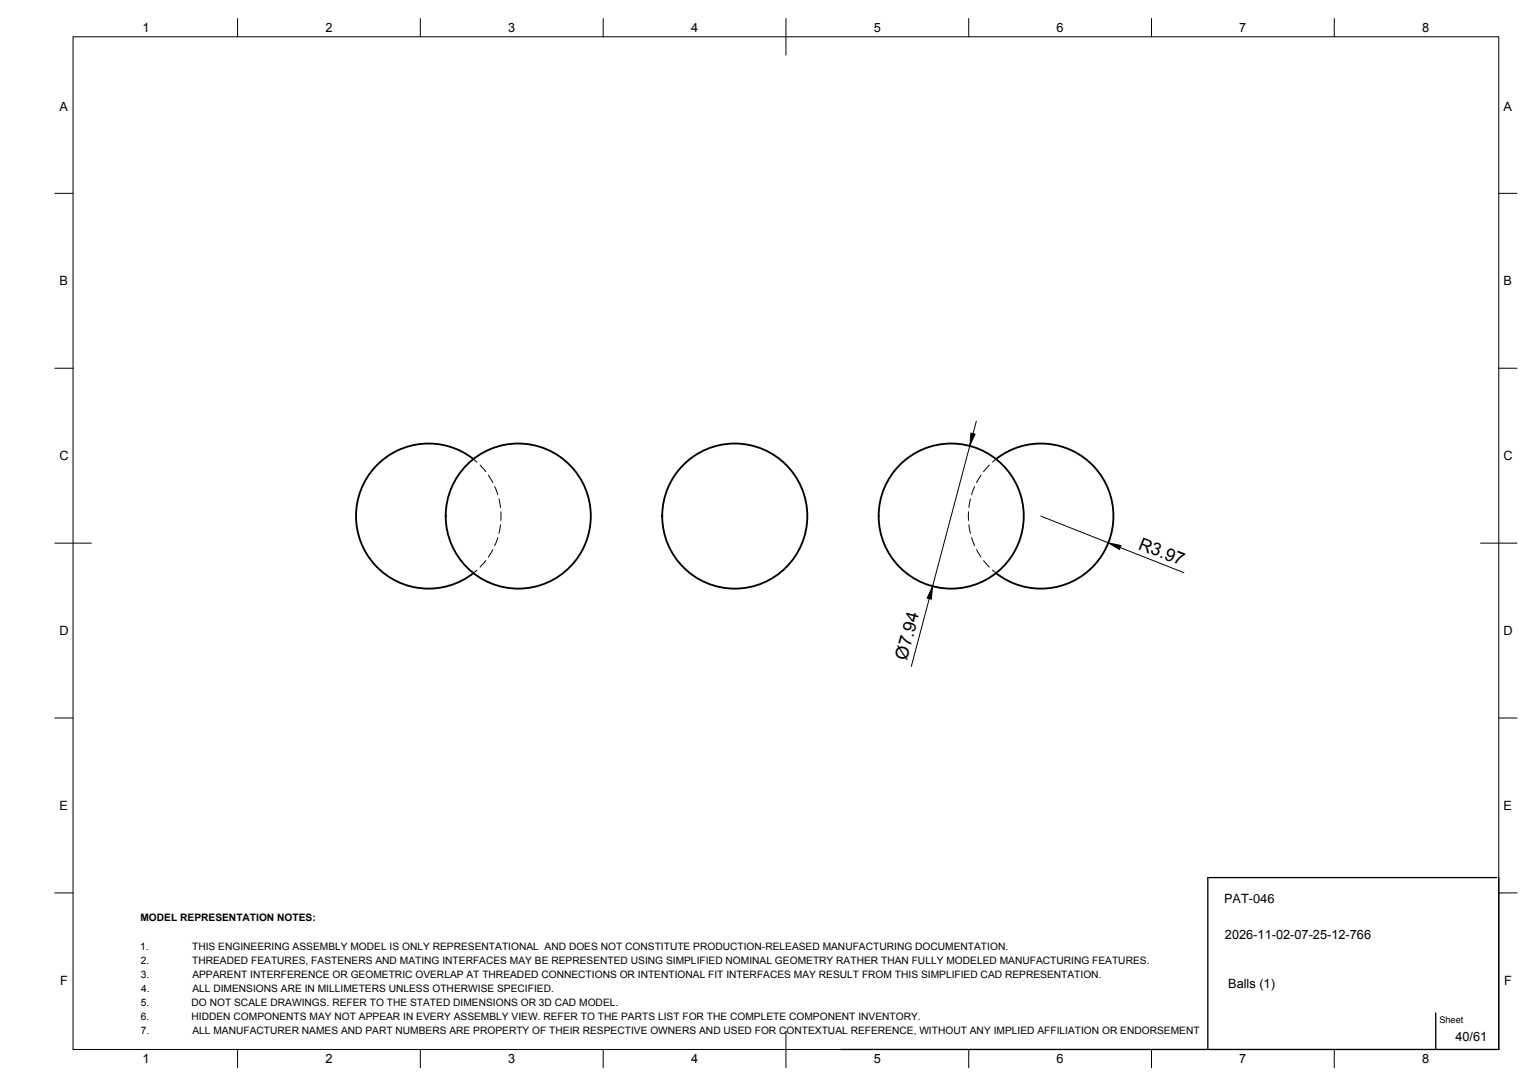
ISO-10303-21;
HEADER;
/* Generated by software containing ST-Developer
 * from STEP Tools, Inc. (www.steptools.com) 
 */

FILE_DESCRIPTION(
/* description */ ('Gear mesh backlash fixture'),
/* implementation_level */ '2;1');

FILE_NAME(
/* name */ 'Balls (1).step',
/* time_stamp */ '2026-10-28T03:26:00-07:00',
/* author */ (''),
/* organization */ (''),
/* preprocessor_version */ 'ST-DEVELOPER v20.2',
/* originating_system */ 'Autodesk Translation Framework v15.17.0.0',
/* authorisation */ '');

FILE_SCHEMA (('AUTOMOTIVE_DESIGN { 1 0 10303 214 3 1 1 }'));
ENDSEC;

DATA;
#10=MECHANICAL_DESIGN_GEOMETRIC_PRESENTATION_REPRESENTATION('',(#1053,#1054,#1055,#1056,#1057,#1058,#1059,#1060),#57900);
#743=SPHERICAL_SURFACE('',#14949,0.3969);
#744=SPHERICAL_SURFACE('',#14951,0.3969);
#745=SPHERICAL_SURFACE('',#14953,0.3969);
#746=SPHERICAL_SURFACE('',#14955,0.3969);
#747=SPHERICAL_SURFACE('',#14957,0.3969);
#748=SPHERICAL_SURFACE('',#14959,0.3969);
#749=SPHERICAL_SURFACE('',#14961,0.3969);
#750=SPHERICAL_SURFACE('',#14963,0.3969);
#946=SHAPE_REPRESENTATION_RELATIONSHIP('SRR','None',#58145,#996);
#996=ADVANCED_BREP_SHAPE_REPRESENTATION('',(#1116,#1117,#1118,#1119,#1120,
#1121,#1122,#1123),#57878);
#1053=STYLED_ITEM('',(#58465),#1116);
#1054=STYLED_ITEM('',(#58465),#1117);
#1055=STYLED_ITEM('',(#58465),#1118);
#1056=STYLED_ITEM('',(#58465),#1119);
#1057=STYLED_ITEM('',(#58465),#1120);
#1058=STYLED_ITEM('',(#58465),#1121);
#1059=STYLED_ITEM('',(#58465),#1122);
#1060=STYLED_ITEM('',(#58465),#1123);
#1116=MANIFOLD_SOLID_BREP('Body1',#13615);
#1117=MANIFOLD_SOLID_BREP('Body2',#13616);
#1118=MANIFOLD_SOLID_BREP('Body3',#13617);
#1119=MANIFOLD_SOLID_BREP('Body4',#13618);
#1120=MANIFOLD_SOLID_BREP('Body5',#13619);
#1121=MANIFOLD_SOLID_BREP('Body6',#13620);
#1122=MANIFOLD_SOLID_BREP('Body7',#13621);
#1123=MANIFOLD_SOLID_BREP('Body8',#13622);
#2060=FACE_OUTER_BOUND('',#2968,.T.);
#2061=FACE_OUTER_BOUND('',#2969,.T.);
#2062=FACE_OUTER_BOUND('',#2970,.T.);
#2063=FACE_OUTER_BOUND('',#2971,.T.);
#2064=FACE_OUTER_BOUND('',#2972,.T.);
#2065=FACE_OUTER_BOUND('',#2973,.T.);
#2066=FACE_OUTER_BOUND('',#2974,.T.);
#2067=FACE_OUTER_BOUND('',#2975,.T.);
#2968=EDGE_LOOP('',(#10539,#10540));
#2969=EDGE_LOOP('',(#10541,#10542));
#2970=EDGE_LOOP('',(#10543,#10544));
#2971=EDGE_LOOP('',(#10545,#10546));
#2972=EDGE_LOOP('',(#10547,#10548));
#2973=EDGE_LOOP('',(#10549,#10550));
#2974=EDGE_LOOP('',(#10551,#10552));
#2975=EDGE_LOOP('',(#10553,#10554));
#5532=CIRCLE('',#14950,0.3969);
#5533=CIRCLE('',#14952,0.3969);
#5534=CIRCLE('',#14954,0.3969);
#5535=CIRCLE('',#14956,0.3969);
#5536=CIRCLE('',#14958,0.3969);
#5537=CIRCLE('',#14960,0.3969);
#5538=CIRCLE('',#14962,0.3969);
#5539=CIRCLE('',#14964,0.3969);
#6334=VERTEX_POINT('',#21485);
#6335=VERTEX_POINT('',#21486);
#6336=VERTEX_POINT('',#21489);
#6337=VERTEX_POINT('',#21490);
#6338=VERTEX_POINT('',#21493);
#6339=VERTEX_POINT('',#21494);
#6340=VERTEX_POINT('',#21497);
#6341=VERTEX_POINT('',#21498);
#6342=VERTEX_POINT('',#21501);
#6343=VERTEX_POINT('',#21502);
#6344=VERTEX_POINT('',#21505);
#6345=VERTEX_POINT('',#21506);
#6346=VERTEX_POINT('',#21509);
#6347=VERTEX_POINT('',#21510);
#6348=VERTEX_POINT('',#21513);
#6349=VERTEX_POINT('',#21514);
#7856=EDGE_CURVE('',#6334,#6335,#5532,.T.);
#7857=EDGE_CURVE('',#6336,#6337,#5533,.T.);
#7858=EDGE_CURVE('',#6338,#6339,#5534,.T.);
#7859=EDGE_CURVE('',#6340,#6341,#5535,.T.);
#7860=EDGE_CURVE('',#6342,#6343,#5536,.T.);
#7861=EDGE_CURVE('',#6344,#6345,#5537,.T.);
#7862=EDGE_CURVE('',#6346,#6347,#5538,.T.);
#7863=EDGE_CURVE('',#6348,#6349,#5539,.T.);
#10539=ORIENTED_EDGE('',*,*,#7856,.T.);
#10540=ORIENTED_EDGE('',*,*,#7856,.F.);
#10541=ORIENTED_EDGE('',*,*,#7857,.T.);
#10542=ORIENTED_EDGE('',*,*,#7857,.F.);
#10543=ORIENTED_EDGE('',*,*,#7858,.T.);
#10544=ORIENTED_EDGE('',*,*,#7858,.F.);
#10545=ORIENTED_EDGE('',*,*,#7859,.T.);
#10546=ORIENTED_EDGE('',*,*,#7859,.F.);
#10547=ORIENTED_EDGE('',*,*,#7860,.T.);
#10548=ORIENTED_EDGE('',*,*,#7860,.F.);
#10549=ORIENTED_EDGE('',*,*,#7861,.T.);
#10550=ORIENTED_EDGE('',*,*,#7861,.F.);
#10551=ORIENTED_EDGE('',*,*,#7862,.T.);
#10552=ORIENTED_EDGE('',*,*,#7862,.F.);
#10553=ORIENTED_EDGE('',*,*,#7863,.T.);
#10554=ORIENTED_EDGE('',*,*,#7863,.F.);
#13177=ADVANCED_FACE('',(#2060),#743,.T.);
#13178=ADVANCED_FACE('',(#2061),#744,.T.);
#13179=ADVANCED_FACE('',(#2062),#745,.T.);
#13180=ADVANCED_FACE('',(#2063),#746,.T.);
#13181=ADVANCED_FACE('',(#2064),#747,.T.);
#13182=ADVANCED_FACE('',(#2065),#748,.T.);
#13183=ADVANCED_FACE('',(#2066),#749,.T.);
#13184=ADVANCED_FACE('',(#2067),#750,.T.);
#13615=CLOSED_SHELL('',(#13177));
#13616=CLOSED_SHELL('',(#13178));
#13617=CLOSED_SHELL('',(#13179));
#13618=CLOSED_SHELL('',(#13180));
#13619=CLOSED_SHELL('',(#13181));
#13620=CLOSED_SHELL('',(#13182));
#13621=CLOSED_SHELL('',(#13183));
#13622=CLOSED_SHELL('',(#13184));
#14948=AXIS2_PLACEMENT_3D('',#21483,#17546,#17547);
#14949=AXIS2_PLACEMENT_3D('',#21484,#17548,#17549);
#14950=AXIS2_PLACEMENT_3D('',#21487,#17550,#17551);
#14951=AXIS2_PLACEMENT_3D('',#21488,#17552,#17553);
#14952=AXIS2_PLACEMENT_3D('',#21491,#17554,#17555);
#14953=AXIS2_PLACEMENT_3D('',#21492,#17556,#17557);
#14954=AXIS2_PLACEMENT_3D('',#21495,#17558,#17559);
#14955=AXIS2_PLACEMENT_3D('',#21496,#17560,#17561);
#14956=AXIS2_PLACEMENT_3D('',#21499,#17562,#17563);
#14957=AXIS2_PLACEMENT_3D('',#21500,#17564,#17565);
#14958=AXIS2_PLACEMENT_3D('',#21503,#17566,#17567);
#14959=AXIS2_PLACEMENT_3D('',#21504,#17568,#17569);
#14960=AXIS2_PLACEMENT_3D('',#21507,#17570,#17571);
#14961=AXIS2_PLACEMENT_3D('',#21508,#17572,#17573);
#14962=AXIS2_PLACEMENT_3D('',#21511,#17574,#17575);
#14963=AXIS2_PLACEMENT_3D('',#21512,#17576,#17577);
#14964=AXIS2_PLACEMENT_3D('',#21515,#17578,#17579);
#17546=DIRECTION('axis',(0.,0.,1.));
#17547=DIRECTION('refdir',(1.,0.,0.));
#17548=DIRECTION('center_axis',(0.,0.,1.));
#17549=DIRECTION('ref_axis',(1.,0.,0.));
#17550=DIRECTION('center_axis',(1.22464679914735E-16,-1.,0.));
#17551=DIRECTION('ref_axis',(-1.,-1.22464679914735E-16,0.));
#17552=DIRECTION('center_axis',(0.707106781186548,0.,0.707106781186548));
#17553=DIRECTION('ref_axis',(0.707106781186548,0.,-0.707106781186548));
#17554=DIRECTION('center_axis',(8.65956056235493E-17,-1.,-8.65956056235493E-17));
#17555=DIRECTION('ref_axis',(-0.707106781186548,-1.22464679914735E-16,0.707106781186548));
#17556=DIRECTION('center_axis',(1.,0.,0.));
#17557=DIRECTION('ref_axis',(6.12323399573677E-17,0.,-1.));
#17558=DIRECTION('center_axis',(7.49879891330929E-33,-1.,-1.22464679914735E-16));
#17559=DIRECTION('ref_axis',(-6.12323399573677E-17,-1.22464679914735E-16,
1.));
#17560=DIRECTION('center_axis',(0.707106781186548,0.,-0.707106781186548));
#17561=DIRECTION('ref_axis',(-0.707106781186548,0.,-0.707106781186548));
#17562=DIRECTION('center_axis',(-8.65956056235493E-17,-1.,-8.65956056235493E-17));
#17563=DIRECTION('ref_axis',(0.707106781186548,-1.22464679914735E-16,0.707106781186548));
#17564=DIRECTION('center_axis',(0.,0.,-1.));
#17565=DIRECTION('ref_axis',(-1.,0.,-1.22464679914735E-16));
#17566=DIRECTION('center_axis',(-1.22464679914735E-16,-1.,-1.49975978266186E-32));
#17567=DIRECTION('ref_axis',(1.,-1.22464679914735E-16,1.22464679914735E-16));
#17568=DIRECTION('center_axis',(-0.707106781186548,0.,-0.707106781186548));
#17569=DIRECTION('ref_axis',(-0.707106781186548,0.,0.707106781186548));
#17570=DIRECTION('center_axis',(-8.65956056235493E-17,-1.,8.65956056235493E-17));
#17571=DIRECTION('ref_axis',(0.707106781186548,-1.22464679914735E-16,-0.707106781186548));
#17572=DIRECTION('center_axis',(-1.,0.,0.));
#17573=DIRECTION('ref_axis',(-1.83697019872103E-16,0.,1.));
#17574=DIRECTION('center_axis',(-2.24963967399279E-32,-1.,1.22464679914735E-16));
#17575=DIRECTION('ref_axis',(1.83697019872103E-16,-1.22464679914735E-16,
-1.));
#17576=DIRECTION('center_axis',(-0.707106781186548,0.,0.707106781186548));
#17577=DIRECTION('ref_axis',(0.707106781186548,0.,0.707106781186548));
#17578=DIRECTION('center_axis',(8.65956056235493E-17,-1.,8.65956056235494E-17));
#17579=DIRECTION('ref_axis',(-0.707106781186548,-1.22464679914735E-16,-0.707106781186548));
#21483=CARTESIAN_POINT('',(0.,0.,0.));
#21484=CARTESIAN_POINT('Origin',(1.675,0.,0.));
#21485=CARTESIAN_POINT('',(1.675,-2.97627328869245E-33,0.3969));
#21486=CARTESIAN_POINT('',(1.675,-2.97627328869245E-33,-0.3969));
#21487=CARTESIAN_POINT('Origin',(1.675,0.,0.));
#21488=CARTESIAN_POINT('Origin',(1.18440385848747,0.,-1.18440385848747));
#21489=CARTESIAN_POINT('',(1.46505453994041,3.1867025333467E-33,-0.903753177034526));
#21490=CARTESIAN_POINT('',(0.903753177034527,-9.13924911073161E-33,-1.46505453994041));
#21491=CARTESIAN_POINT('Origin',(1.18440385848747,0.,-1.18440385848747));
#21492=CARTESIAN_POINT('Origin',(1.02564169428591E-16,0.,-1.675));
#21493=CARTESIAN_POINT('',(0.3969,-2.97627328869246E-33,-1.675));
#21494=CARTESIAN_POINT('',(-0.3969,-2.97627328869245E-33,-1.675));
#21495=CARTESIAN_POINT('Origin',(1.02564169428591E-16,0.,-1.675));
#21496=CARTESIAN_POINT('Origin',(-1.18440385848747,0.,-1.18440385848747));
#21497=CARTESIAN_POINT('',(-0.903753177034526,3.1867025333467E-33,-1.46505453994041));
#21498=CARTESIAN_POINT('',(-1.46505453994041,-9.13924911073161E-33,-0.903753177034527));
#21499=CARTESIAN_POINT('Origin',(-1.18440385848747,0.,-1.18440385848747));
#21500=CARTESIAN_POINT('Origin',(-1.675,0.,-2.05128338857182E-16));
#21501=CARTESIAN_POINT('',(-1.675,-2.97627328869246E-33,-0.3969));
#21502=CARTESIAN_POINT('',(-1.675,-2.97627328869245E-33,0.3969));
#21503=CARTESIAN_POINT('Origin',(-1.675,0.,-2.05128338857182E-16));
#21504=CARTESIAN_POINT('Origin',(-1.18440385848747,0.,1.18440385848747));
#21505=CARTESIAN_POINT('',(-1.46505453994041,6.26819044436628E-33,0.903753177034526));
#21506=CARTESIAN_POINT('',(-0.903753177034527,-1.22207370217512E-32,1.46505453994041));
#21507=CARTESIAN_POINT('Origin',(-1.18440385848747,0.,1.18440385848747));
#21508=CARTESIAN_POINT('Origin',(-3.07692508285772E-16,0.,1.675));
#21509=CARTESIAN_POINT('',(-0.3969,-2.97627328869246E-33,1.675));
#21510=CARTESIAN_POINT('',(0.396899999999999,-2.97627328869245E-33,1.675));
#21511=CARTESIAN_POINT('Origin',(-3.07692508285772E-16,0.,1.675));
#21512=CARTESIAN_POINT('Origin',(1.18440385848747,0.,1.18440385848747));
#21513=CARTESIAN_POINT('',(0.903753177034526,9.34967835538585E-33,1.46505453994041));
#21514=CARTESIAN_POINT('',(1.46505453994041,-1.53022249327708E-32,0.903753177034527));
#21515=CARTESIAN_POINT('Origin',(1.18440385848747,0.,1.18440385848747));
#57819=UNCERTAINTY_MEASURE_WITH_UNIT(LENGTH_MEASURE(0.001),#57901,
'DISTANCE_ACCURACY_VALUE',
'Maximum model space distance between geometric entities at asserted c
onnectivities');
#57841=UNCERTAINTY_MEASURE_WITH_UNIT(LENGTH_MEASURE(0.001),#57901,
'DISTANCE_ACCURACY_VALUE',
'Maximum model space distance between geometric entities at asserted c
onnectivities');
#57878=(
GEOMETRIC_REPRESENTATION_CONTEXT(3)
GLOBAL_UNCERTAINTY_ASSIGNED_CONTEXT((#57819))
GLOBAL_UNIT_ASSIGNED_CONTEXT((#57901,#57903,#57904))
REPRESENTATION_CONTEXT('','3D')
);
#57900=(
GEOMETRIC_REPRESENTATION_CONTEXT(3)
GLOBAL_UNCERTAINTY_ASSIGNED_CONTEXT((#57841))
GLOBAL_UNIT_ASSIGNED_CONTEXT((#57901,#57903,#57904))
REPRESENTATION_CONTEXT('','3D')
);
#57901=(
LENGTH_UNIT()
NAMED_UNIT(*)
SI_UNIT(.CENTI.,.METRE.)
);
#57903=(
NAMED_UNIT(*)
PLANE_ANGLE_UNIT()
SI_UNIT($,.RADIAN.)
);
#57904=(
NAMED_UNIT(*)
SI_UNIT($,.STERADIAN.)
SOLID_ANGLE_UNIT()
);
#57941=SHAPE_DEFINITION_REPRESENTATION(#58007,#58145);
#58007=PRODUCT_DEFINITION_SHAPE('',$,#58204);
#58145=SHAPE_REPRESENTATION('',(#14948),#57878);
#58167=PRODUCT_DEFINITION_CONTEXT('part definition',#58343,'design');
#58204=PRODUCT_DEFINITION('Balls (1)','Balls (1)',#58262,#58167);
#58262=PRODUCT_DEFINITION_FORMATION('',$,#58381);
#58343=APPLICATION_CONTEXT(
'Core Data for Automotive Mechanical Design Process');
#58344=PRODUCT_CONTEXT('part definition',#58343,'mechanical');
#58381=PRODUCT('Balls (1)','Balls (1)','Balls (1)',(#58344));
#58459=COLOUR_RGB('Grey',0.48,0.52,0.57);
#58460=FILL_AREA_STYLE_COLOUR('',#58459);
#58461=FILL_AREA_STYLE('',(#58460));
#58462=SURFACE_STYLE_FILL_AREA(#58461);
#58463=SURFACE_SIDE_STYLE('',(#58462));
#58464=SURFACE_STYLE_USAGE(.BOTH.,#58463);
#58465=PRESENTATION_STYLE_ASSIGNMENT((#58464));
ENDSEC;
END-ISO-10303-21;
